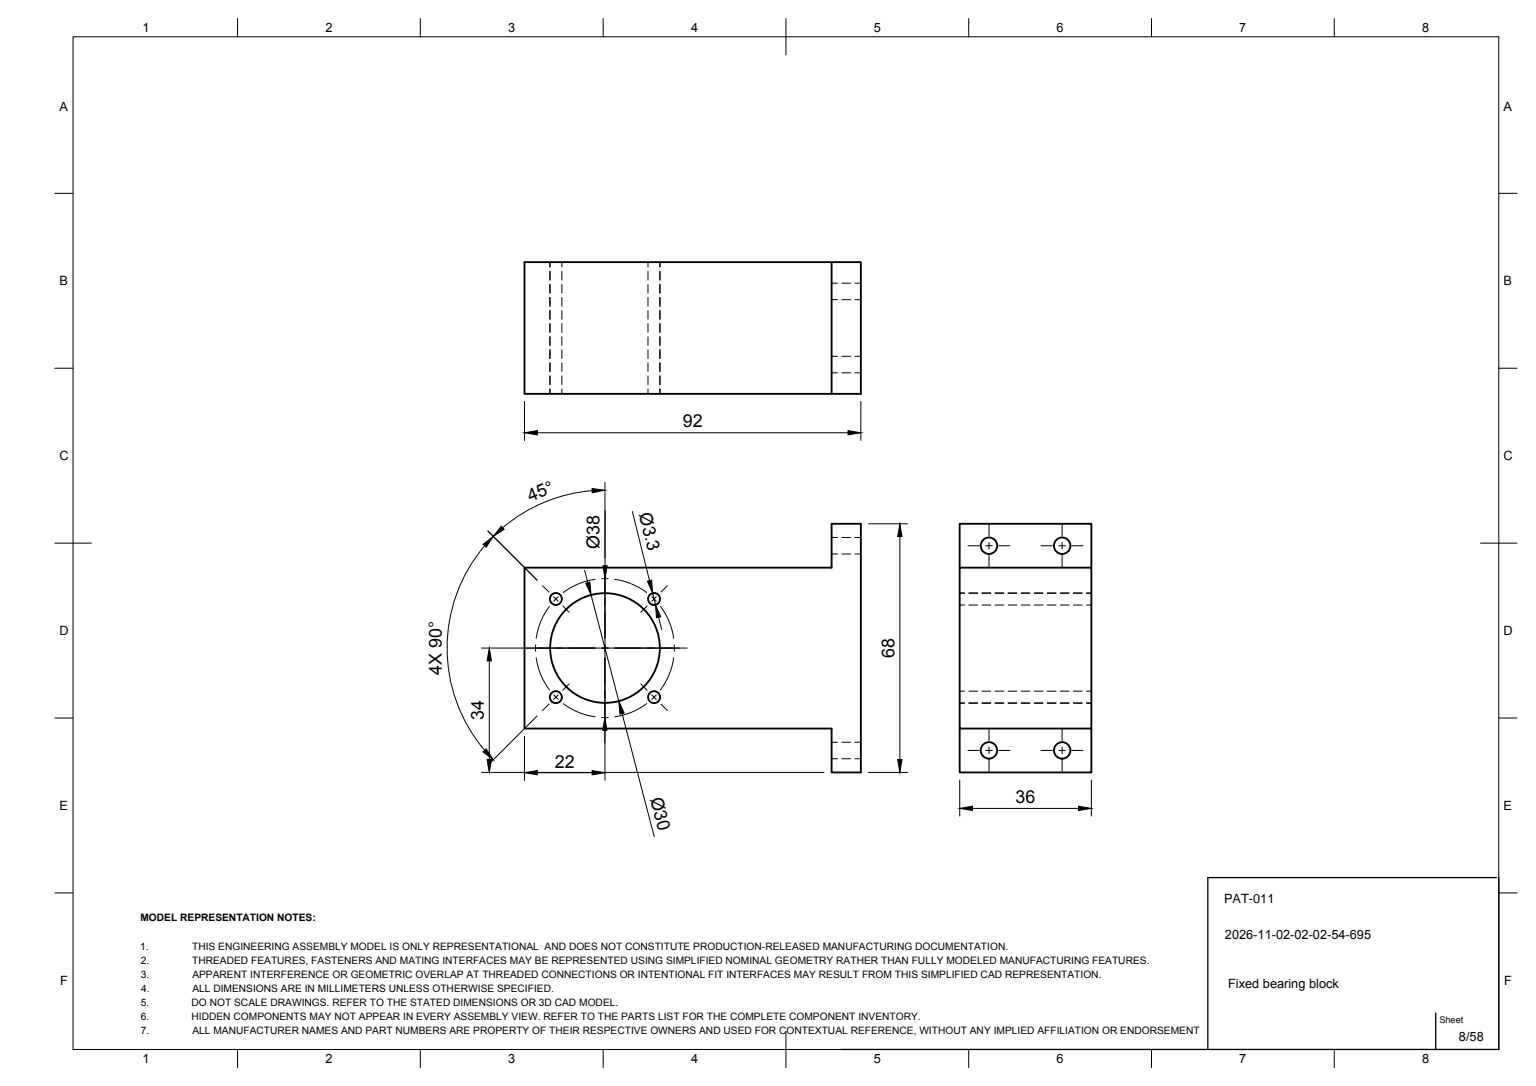
ISO-10303-21;
HEADER;
/* Generated by software containing ST-Developer
 * from STEP Tools, Inc. (www.steptools.com) 
 */

FILE_DESCRIPTION(
/* description */ ('Belt tension measurement rig'),
/* implementation_level */ '2;1');

FILE_NAME(
/* name */ 'Fixed bearing block.step',
/* time_stamp */ '2026-10-28T03:24:44-07:00',
/* author */ (''),
/* organization */ (''),
/* preprocessor_version */ 'ST-DEVELOPER v20.2',
/* originating_system */ 'Autodesk Translation Framework v15.17.0.0',
/* authorisation */ '');

FILE_SCHEMA (('AUTOMOTIVE_DESIGN { 1 0 10303 214 3 1 1 }'));
ENDSEC;

DATA;
#10=MECHANICAL_DESIGN_GEOMETRIC_PRESENTATION_REPRESENTATION('',(#695),#23587);
#585=SHAPE_REPRESENTATION_RELATIONSHIP('SRR','None',#23830,#640);
#640=ADVANCED_BREP_SHAPE_REPRESENTATION('',(#765),#23528);
#695=STYLED_ITEM('',(#24211),#765);
#765=MANIFOLD_SOLID_BREP('Body1',#12200);
#843=FACE_BOUND('',#2126,.T.);
#844=FACE_BOUND('',#2127,.T.);
#845=FACE_BOUND('',#2129,.T.);
#846=FACE_BOUND('',#2130,.T.);
#847=FACE_BOUND('',#2134,.T.);
#848=FACE_BOUND('',#2135,.T.);
#849=FACE_BOUND('',#2136,.T.);
#850=FACE_BOUND('',#2137,.T.);
#851=FACE_BOUND('',#2138,.T.);
#852=FACE_BOUND('',#2141,.T.);
#853=FACE_BOUND('',#2142,.T.);
#854=FACE_BOUND('',#2143,.T.);
#855=FACE_BOUND('',#2144,.T.);
#856=FACE_BOUND('',#2145,.T.);
#857=FACE_BOUND('',#2149,.T.);
#858=FACE_BOUND('',#2150,.T.);
#859=FACE_BOUND('',#2151,.T.);
#860=FACE_BOUND('',#2152,.T.);
#1069=PLANE('',#12983);
#1070=PLANE('',#12984);
#1071=PLANE('',#12985);
#1072=PLANE('',#12986);
#1073=PLANE('',#12987);
#1074=PLANE('',#12988);
#1075=PLANE('',#12989);
#1076=PLANE('',#12990);
#1077=PLANE('',#12991);
#1078=PLANE('',#12992);
#1398=FACE_OUTER_BOUND('',#2116,.T.);
#1399=FACE_OUTER_BOUND('',#2117,.T.);
#1400=FACE_OUTER_BOUND('',#2118,.T.);
#1401=FACE_OUTER_BOUND('',#2119,.T.);
#1402=FACE_OUTER_BOUND('',#2120,.T.);
#1403=FACE_OUTER_BOUND('',#2121,.T.);
#1404=FACE_OUTER_BOUND('',#2122,.T.);
#1405=FACE_OUTER_BOUND('',#2123,.T.);
#1406=FACE_OUTER_BOUND('',#2124,.T.);
#1407=FACE_OUTER_BOUND('',#2125,.T.);
#1408=FACE_OUTER_BOUND('',#2128,.T.);
#1409=FACE_OUTER_BOUND('',#2131,.T.);
#1410=FACE_OUTER_BOUND('',#2132,.T.);
#1411=FACE_OUTER_BOUND('',#2133,.T.);
#1412=FACE_OUTER_BOUND('',#2139,.T.);
#1413=FACE_OUTER_BOUND('',#2140,.T.);
#1414=FACE_OUTER_BOUND('',#2146,.T.);
#1415=FACE_OUTER_BOUND('',#2147,.T.);
#1416=FACE_OUTER_BOUND('',#2148,.T.);
#2116=EDGE_LOOP('',(#8094,#8095,#8096,#8097));
#2117=EDGE_LOOP('',(#8098,#8099,#8100,#8101));
#2118=EDGE_LOOP('',(#8102,#8103,#8104,#8105));
#2119=EDGE_LOOP('',(#8106,#8107,#8108,#8109));
#2120=EDGE_LOOP('',(#8110,#8111,#8112,#8113));
#2121=EDGE_LOOP('',(#8114,#8115,#8116,#8117));
#2122=EDGE_LOOP('',(#8118,#8119,#8120,#8121));
#2123=EDGE_LOOP('',(#8122,#8123,#8124,#8125));
#2124=EDGE_LOOP('',(#8126,#8127,#8128,#8129));
#2125=EDGE_LOOP('',(#8130,#8131,#8132,#8133));
#2126=EDGE_LOOP('',(#8134));
#2127=EDGE_LOOP('',(#8135));
#2128=EDGE_LOOP('',(#8136,#8137,#8138,#8139));
#2129=EDGE_LOOP('',(#8140));
#2130=EDGE_LOOP('',(#8141));
#2131=EDGE_LOOP('',(#8142,#8143,#8144,#8145));
#2132=EDGE_LOOP('',(#8146,#8147,#8148,#8149));
#2133=EDGE_LOOP('',(#8150,#8151,#8152,#8153,#8154,#8155,#8156,#8157));
#2134=EDGE_LOOP('',(#8158));
#2135=EDGE_LOOP('',(#8159));
#2136=EDGE_LOOP('',(#8160));
#2137=EDGE_LOOP('',(#8161));
#2138=EDGE_LOOP('',(#8162));
#2139=EDGE_LOOP('',(#8163,#8164,#8165,#8166));
#2140=EDGE_LOOP('',(#8167,#8168,#8169,#8170,#8171,#8172,#8173,#8174));
#2141=EDGE_LOOP('',(#8175));
#2142=EDGE_LOOP('',(#8176));
#2143=EDGE_LOOP('',(#8177));
#2144=EDGE_LOOP('',(#8178));
#2145=EDGE_LOOP('',(#8179));
#2146=EDGE_LOOP('',(#8180,#8181,#8182,#8183));
#2147=EDGE_LOOP('',(#8184,#8185,#8186,#8187));
#2148=EDGE_LOOP('',(#8188,#8189,#8190,#8191));
#2149=EDGE_LOOP('',(#8192));
#2150=EDGE_LOOP('',(#8193));
#2151=EDGE_LOOP('',(#8194));
#2152=EDGE_LOOP('',(#8195));
#3018=LINE('',#18736,#3769);
#3019=LINE('',#18742,#3770);
#3020=LINE('',#18748,#3771);
#3021=LINE('',#18754,#3772);
#3022=LINE('',#18760,#3773);
#3023=LINE('',#18766,#3774);
#3024=LINE('',#18772,#3775);
#3025=LINE('',#18778,#3776);
#3026=LINE('',#18784,#3777);
#3027=LINE('',#18789,#3778);
#3028=LINE('',#18791,#3779);
#3029=LINE('',#18793,#3780);
#3030=LINE('',#18794,#3781);
#3031=LINE('',#18798,#3782);
#3032=LINE('',#18800,#3783);
#3033=LINE('',#18802,#3784);
#3034=LINE('',#18803,#3785);
#3035=LINE('',#18806,#3786);
#3036=LINE('',#18808,#3787);
#3037=LINE('',#18809,#3788);
#3038=LINE('',#18812,#3789);
#3039=LINE('',#18814,#3790);
#3040=LINE('',#18815,#3791);
#3041=LINE('',#18818,#3792);
#3042=LINE('',#18820,#3793);
#3043=LINE('',#18821,#3794);
#3044=LINE('',#18822,#3795);
#3045=LINE('',#18825,#3796);
#3046=LINE('',#18826,#3797);
#3047=LINE('',#18829,#3798);
#3048=LINE('',#18830,#3799);
#3049=LINE('',#18831,#3800);
#3050=LINE('',#18833,#3801);
#3769=VECTOR('',#14731,0.165);
#3770=VECTOR('',#14738,0.165);
#3771=VECTOR('',#14745,0.165);
#3772=VECTOR('',#14752,0.165);
#3773=VECTOR('',#14759,1.5);
#3774=VECTOR('',#14766,0.225);
#3775=VECTOR('',#14773,0.225);
#3776=VECTOR('',#14780,0.225);
#3777=VECTOR('',#14787,0.225);
#3778=VECTOR('',#14792,1.);
#3779=VECTOR('',#14793,1.);
#3780=VECTOR('',#14794,1.);
#3781=VECTOR('',#14795,1.);
#3782=VECTOR('',#14798,1.);
#3783=VECTOR('',#14799,1.);
#3784=VECTOR('',#14800,1.);
#3785=VECTOR('',#14801,1.);
#3786=VECTOR('',#14804,1.);
#3787=VECTOR('',#14805,1.);
#3788=VECTOR('',#14806,1.);
#3789=VECTOR('',#14809,1.);
#3790=VECTOR('',#14810,1.);
#3791=VECTOR('',#14811,1.);
#3792=VECTOR('',#14814,1.);
#3793=VECTOR('',#14815,1.);
#3794=VECTOR('',#14816,1.);
#3795=VECTOR('',#14817,1.);
#3796=VECTOR('',#14820,1.);
#3797=VECTOR('',#14821,1.);
#3798=VECTOR('',#14824,1.);
#3799=VECTOR('',#14825,1.);
#3800=VECTOR('',#14826,1.);
#3801=VECTOR('',#14829,1.);
#4498=CIRCLE('',#12957,0.165);
#4499=CIRCLE('',#12958,0.165);
#4500=CIRCLE('',#12960,0.165);
#4501=CIRCLE('',#12961,0.165);
#4502=CIRCLE('',#12963,0.165);
#4503=CIRCLE('',#12964,0.165);
#4504=CIRCLE('',#12966,0.165);
#4505=CIRCLE('',#12967,0.165);
#4506=CIRCLE('',#12969,1.5);
#4507=CIRCLE('',#12970,1.5);
#4508=CIRCLE('',#12972,0.225);
#4509=CIRCLE('',#12973,0.225);
#4510=CIRCLE('',#12975,0.225);
#4511=CIRCLE('',#12976,0.225);
#4512=CIRCLE('',#12978,0.225);
#4513=CIRCLE('',#12979,0.225);
#4514=CIRCLE('',#12981,0.225);
#4515=CIRCLE('',#12982,0.225);
#5290=VERTEX_POINT('',#18733);
#5291=VERTEX_POINT('',#18735);
#5292=VERTEX_POINT('',#18739);
#5293=VERTEX_POINT('',#18741);
#5294=VERTEX_POINT('',#18745);
#5295=VERTEX_POINT('',#18747);
#5296=VERTEX_POINT('',#18751);
#5297=VERTEX_POINT('',#18753);
#5298=VERTEX_POINT('',#18757);
#5299=VERTEX_POINT('',#18759);
#5300=VERTEX_POINT('',#18763);
#5301=VERTEX_POINT('',#18765);
#5302=VERTEX_POINT('',#18769);
#5303=VERTEX_POINT('',#18771);
#5304=VERTEX_POINT('',#18775);
#5305=VERTEX_POINT('',#18777);
#5306=VERTEX_POINT('',#18781);
#5307=VERTEX_POINT('',#18783);
#5308=VERTEX_POINT('',#18787);
#5309=VERTEX_POINT('',#18788);
#5310=VERTEX_POINT('',#18790);
#5311=VERTEX_POINT('',#18792);
#5312=VERTEX_POINT('',#18796);
#5313=VERTEX_POINT('',#18797);
#5314=VERTEX_POINT('',#18799);
#5315=VERTEX_POINT('',#18801);
#5316=VERTEX_POINT('',#18805);
#5317=VERTEX_POINT('',#18807);
#5318=VERTEX_POINT('',#18811);
#5319=VERTEX_POINT('',#18813);
#5320=VERTEX_POINT('',#18817);
#5321=VERTEX_POINT('',#18819);
#5322=VERTEX_POINT('',#18824);
#5323=VERTEX_POINT('',#18828);
#6406=EDGE_CURVE('',#5290,#5290,#4498,.T.);
#6407=EDGE_CURVE('',#5290,#5291,#3018,.T.);
#6408=EDGE_CURVE('',#5291,#5291,#4499,.T.);
#6409=EDGE_CURVE('',#5292,#5292,#4500,.T.);
#6410=EDGE_CURVE('',#5292,#5293,#3019,.T.);
#6411=EDGE_CURVE('',#5293,#5293,#4501,.T.);
#6412=EDGE_CURVE('',#5294,#5294,#4502,.T.);
#6413=EDGE_CURVE('',#5294,#5295,#3020,.T.);
#6414=EDGE_CURVE('',#5295,#5295,#4503,.T.);
#6415=EDGE_CURVE('',#5296,#5296,#4504,.T.);
#6416=EDGE_CURVE('',#5296,#5297,#3021,.T.);
#6417=EDGE_CURVE('',#5297,#5297,#4505,.T.);
#6418=EDGE_CURVE('',#5298,#5298,#4506,.T.);
#6419=EDGE_CURVE('',#5298,#5299,#3022,.T.);
#6420=EDGE_CURVE('',#5299,#5299,#4507,.T.);
#6421=EDGE_CURVE('',#5300,#5300,#4508,.T.);
#6422=EDGE_CURVE('',#5300,#5301,#3023,.T.);
#6423=EDGE_CURVE('',#5301,#5301,#4509,.T.);
#6424=EDGE_CURVE('',#5302,#5302,#4510,.T.);
#6425=EDGE_CURVE('',#5302,#5303,#3024,.T.);
#6426=EDGE_CURVE('',#5303,#5303,#4511,.T.);
#6427=EDGE_CURVE('',#5304,#5304,#4512,.T.);
#6428=EDGE_CURVE('',#5304,#5305,#3025,.T.);
#6429=EDGE_CURVE('',#5305,#5305,#4513,.T.);
#6430=EDGE_CURVE('',#5306,#5306,#4514,.T.);
#6431=EDGE_CURVE('',#5306,#5307,#3026,.T.);
#6432=EDGE_CURVE('',#5307,#5307,#4515,.T.);
#6433=EDGE_CURVE('',#5308,#5309,#3027,.T.);
#6434=EDGE_CURVE('',#5310,#5308,#3028,.T.);
#6435=EDGE_CURVE('',#5310,#5311,#3029,.T.);
#6436=EDGE_CURVE('',#5309,#5311,#3030,.T.);
#6437=EDGE_CURVE('',#5312,#5313,#3031,.T.);
#6438=EDGE_CURVE('',#5314,#5312,#3032,.T.);
#6439=EDGE_CURVE('',#5315,#5314,#3033,.T.);
#6440=EDGE_CURVE('',#5313,#5315,#3034,.T.);
#6441=EDGE_CURVE('',#5315,#5316,#3035,.T.);
#6442=EDGE_CURVE('',#5317,#5314,#3036,.T.);
#6443=EDGE_CURVE('',#5316,#5317,#3037,.T.);
#6444=EDGE_CURVE('',#5318,#5310,#3038,.T.);
#6445=EDGE_CURVE('',#5318,#5319,#3039,.T.);
#6446=EDGE_CURVE('',#5311,#5319,#3040,.T.);
#6447=EDGE_CURVE('',#5308,#5320,#3041,.T.);
#6448=EDGE_CURVE('',#5321,#5320,#3042,.T.);
#6449=EDGE_CURVE('',#5313,#5321,#3043,.T.);
#6450=EDGE_CURVE('',#5316,#5318,#3044,.T.);
#6451=EDGE_CURVE('',#5309,#5322,#3045,.T.);
#6452=EDGE_CURVE('',#5320,#5322,#3046,.T.);
#6453=EDGE_CURVE('',#5312,#5323,#3047,.T.);
#6454=EDGE_CURVE('',#5322,#5323,#3048,.T.);
#6455=EDGE_CURVE('',#5319,#5317,#3049,.T.);
#6456=EDGE_CURVE('',#5323,#5321,#3050,.T.);
#8094=ORIENTED_EDGE('',*,*,#6406,.F.);
#8095=ORIENTED_EDGE('',*,*,#6407,.T.);
#8096=ORIENTED_EDGE('',*,*,#6408,.F.);
#8097=ORIENTED_EDGE('',*,*,#6407,.F.);
#8098=ORIENTED_EDGE('',*,*,#6409,.F.);
#8099=ORIENTED_EDGE('',*,*,#6410,.T.);
#8100=ORIENTED_EDGE('',*,*,#6411,.F.);
#8101=ORIENTED_EDGE('',*,*,#6410,.F.);
#8102=ORIENTED_EDGE('',*,*,#6412,.F.);
#8103=ORIENTED_EDGE('',*,*,#6413,.T.);
#8104=ORIENTED_EDGE('',*,*,#6414,.F.);
#8105=ORIENTED_EDGE('',*,*,#6413,.F.);
#8106=ORIENTED_EDGE('',*,*,#6415,.F.);
#8107=ORIENTED_EDGE('',*,*,#6416,.T.);
#8108=ORIENTED_EDGE('',*,*,#6417,.F.);
#8109=ORIENTED_EDGE('',*,*,#6416,.F.);
#8110=ORIENTED_EDGE('',*,*,#6418,.F.);
#8111=ORIENTED_EDGE('',*,*,#6419,.T.);
#8112=ORIENTED_EDGE('',*,*,#6420,.F.);
#8113=ORIENTED_EDGE('',*,*,#6419,.F.);
#8114=ORIENTED_EDGE('',*,*,#6421,.F.);
#8115=ORIENTED_EDGE('',*,*,#6422,.T.);
#8116=ORIENTED_EDGE('',*,*,#6423,.F.);
#8117=ORIENTED_EDGE('',*,*,#6422,.F.);
#8118=ORIENTED_EDGE('',*,*,#6424,.F.);
#8119=ORIENTED_EDGE('',*,*,#6425,.T.);
#8120=ORIENTED_EDGE('',*,*,#6426,.F.);
#8121=ORIENTED_EDGE('',*,*,#6425,.F.);
#8122=ORIENTED_EDGE('',*,*,#6427,.F.);
#8123=ORIENTED_EDGE('',*,*,#6428,.T.);
#8124=ORIENTED_EDGE('',*,*,#6429,.F.);
#8125=ORIENTED_EDGE('',*,*,#6428,.F.);
#8126=ORIENTED_EDGE('',*,*,#6430,.F.);
#8127=ORIENTED_EDGE('',*,*,#6431,.T.);
#8128=ORIENTED_EDGE('',*,*,#6432,.F.);
#8129=ORIENTED_EDGE('',*,*,#6431,.F.);
#8130=ORIENTED_EDGE('',*,*,#6433,.F.);
#8131=ORIENTED_EDGE('',*,*,#6434,.F.);
#8132=ORIENTED_EDGE('',*,*,#6435,.T.);
#8133=ORIENTED_EDGE('',*,*,#6436,.F.);
#8134=ORIENTED_EDGE('',*,*,#6423,.T.);
#8135=ORIENTED_EDGE('',*,*,#6432,.T.);
#8136=ORIENTED_EDGE('',*,*,#6437,.F.);
#8137=ORIENTED_EDGE('',*,*,#6438,.F.);
#8138=ORIENTED_EDGE('',*,*,#6439,.F.);
#8139=ORIENTED_EDGE('',*,*,#6440,.F.);
#8140=ORIENTED_EDGE('',*,*,#6426,.T.);
#8141=ORIENTED_EDGE('',*,*,#6429,.T.);
#8142=ORIENTED_EDGE('',*,*,#6441,.F.);
#8143=ORIENTED_EDGE('',*,*,#6439,.T.);
#8144=ORIENTED_EDGE('',*,*,#6442,.F.);
#8145=ORIENTED_EDGE('',*,*,#6443,.F.);
#8146=ORIENTED_EDGE('',*,*,#6444,.F.);
#8147=ORIENTED_EDGE('',*,*,#6445,.T.);
#8148=ORIENTED_EDGE('',*,*,#6446,.F.);
#8149=ORIENTED_EDGE('',*,*,#6435,.F.);
#8150=ORIENTED_EDGE('',*,*,#6447,.T.);
#8151=ORIENTED_EDGE('',*,*,#6448,.F.);
#8152=ORIENTED_EDGE('',*,*,#6449,.F.);
#8153=ORIENTED_EDGE('',*,*,#6440,.T.);
#8154=ORIENTED_EDGE('',*,*,#6441,.T.);
#8155=ORIENTED_EDGE('',*,*,#6450,.T.);
#8156=ORIENTED_EDGE('',*,*,#6444,.T.);
#8157=ORIENTED_EDGE('',*,*,#6434,.T.);
#8158=ORIENTED_EDGE('',*,*,#6418,.T.);
#8159=ORIENTED_EDGE('',*,*,#6415,.T.);
#8160=ORIENTED_EDGE('',*,*,#6412,.T.);
#8161=ORIENTED_EDGE('',*,*,#6409,.T.);
#8162=ORIENTED_EDGE('',*,*,#6406,.T.);
#8163=ORIENTED_EDGE('',*,*,#6433,.T.);
#8164=ORIENTED_EDGE('',*,*,#6451,.T.);
#8165=ORIENTED_EDGE('',*,*,#6452,.F.);
#8166=ORIENTED_EDGE('',*,*,#6447,.F.);
#8167=ORIENTED_EDGE('',*,*,#6453,.T.);
#8168=ORIENTED_EDGE('',*,*,#6454,.F.);
#8169=ORIENTED_EDGE('',*,*,#6451,.F.);
#8170=ORIENTED_EDGE('',*,*,#6436,.T.);
#8171=ORIENTED_EDGE('',*,*,#6446,.T.);
#8172=ORIENTED_EDGE('',*,*,#6455,.T.);
#8173=ORIENTED_EDGE('',*,*,#6442,.T.);
#8174=ORIENTED_EDGE('',*,*,#6438,.T.);
#8175=ORIENTED_EDGE('',*,*,#6420,.T.);
#8176=ORIENTED_EDGE('',*,*,#6417,.T.);
#8177=ORIENTED_EDGE('',*,*,#6414,.T.);
#8178=ORIENTED_EDGE('',*,*,#6411,.T.);
#8179=ORIENTED_EDGE('',*,*,#6408,.T.);
#8180=ORIENTED_EDGE('',*,*,#6437,.T.);
#8181=ORIENTED_EDGE('',*,*,#6449,.T.);
#8182=ORIENTED_EDGE('',*,*,#6456,.F.);
#8183=ORIENTED_EDGE('',*,*,#6453,.F.);
#8184=ORIENTED_EDGE('',*,*,#6456,.T.);
#8185=ORIENTED_EDGE('',*,*,#6448,.T.);
#8186=ORIENTED_EDGE('',*,*,#6452,.T.);
#8187=ORIENTED_EDGE('',*,*,#6454,.T.);
#8188=ORIENTED_EDGE('',*,*,#6455,.F.);
#8189=ORIENTED_EDGE('',*,*,#6445,.F.);
#8190=ORIENTED_EDGE('',*,*,#6450,.F.);
#8191=ORIENTED_EDGE('',*,*,#6443,.T.);
#8192=ORIENTED_EDGE('',*,*,#6421,.T.);
#8193=ORIENTED_EDGE('',*,*,#6424,.T.);
#8194=ORIENTED_EDGE('',*,*,#6427,.T.);
#8195=ORIENTED_EDGE('',*,*,#6430,.T.);
#11172=CYLINDRICAL_SURFACE('',#12956,0.165);
#11173=CYLINDRICAL_SURFACE('',#12959,0.165);
#11174=CYLINDRICAL_SURFACE('',#12962,0.165);
#11175=CYLINDRICAL_SURFACE('',#12965,0.165);
#11176=CYLINDRICAL_SURFACE('',#12968,1.5);
#11177=CYLINDRICAL_SURFACE('',#12971,0.225);
#11178=CYLINDRICAL_SURFACE('',#12974,0.225);
#11179=CYLINDRICAL_SURFACE('',#12977,0.225);
#11180=CYLINDRICAL_SURFACE('',#12980,0.225);
#11539=ADVANCED_FACE('',(#1398),#11172,.F.);
#11540=ADVANCED_FACE('',(#1399),#11173,.F.);
#11541=ADVANCED_FACE('',(#1400),#11174,.F.);
#11542=ADVANCED_FACE('',(#1401),#11175,.F.);
#11543=ADVANCED_FACE('',(#1402),#11176,.F.);
#11544=ADVANCED_FACE('',(#1403),#11177,.F.);
#11545=ADVANCED_FACE('',(#1404),#11178,.F.);
#11546=ADVANCED_FACE('',(#1405),#11179,.F.);
#11547=ADVANCED_FACE('',(#1406),#11180,.F.);
#11548=ADVANCED_FACE('',(#1407,#843,#844),#1069,.T.);
#11549=ADVANCED_FACE('',(#1408,#845,#846),#1070,.T.);
#11550=ADVANCED_FACE('',(#1409),#1071,.T.);
#11551=ADVANCED_FACE('',(#1410),#1072,.T.);
#11552=ADVANCED_FACE('',(#1411,#847,#848,#849,#850,#851),#1073,.T.);
#11553=ADVANCED_FACE('',(#1412),#1074,.T.);
#11554=ADVANCED_FACE('',(#1413,#852,#853,#854,#855,#856),#1075,.T.);
#11555=ADVANCED_FACE('',(#1414),#1076,.T.);
#11556=ADVANCED_FACE('',(#1415),#1077,.T.);
#11557=ADVANCED_FACE('',(#1416,#857,#858,#859,#860),#1078,.F.);
#12200=CLOSED_SHELL('',(#11539,#11540,#11541,#11542,#11543,#11544,#11545,
#11546,#11547,#11548,#11549,#11550,#11551,#11552,#11553,#11554,#11555,#11556,
#11557));
#12955=AXIS2_PLACEMENT_3D('',#18731,#14725,#14726);
#12956=AXIS2_PLACEMENT_3D('',#18732,#14727,#14728);
#12957=AXIS2_PLACEMENT_3D('',#18734,#14729,#14730);
#12958=AXIS2_PLACEMENT_3D('',#18737,#14732,#14733);
#12959=AXIS2_PLACEMENT_3D('',#18738,#14734,#14735);
#12960=AXIS2_PLACEMENT_3D('',#18740,#14736,#14737);
#12961=AXIS2_PLACEMENT_3D('',#18743,#14739,#14740);
#12962=AXIS2_PLACEMENT_3D('',#18744,#14741,#14742);
#12963=AXIS2_PLACEMENT_3D('',#18746,#14743,#14744);
#12964=AXIS2_PLACEMENT_3D('',#18749,#14746,#14747);
#12965=AXIS2_PLACEMENT_3D('',#18750,#14748,#14749);
#12966=AXIS2_PLACEMENT_3D('',#18752,#14750,#14751);
#12967=AXIS2_PLACEMENT_3D('',#18755,#14753,#14754);
#12968=AXIS2_PLACEMENT_3D('',#18756,#14755,#14756);
#12969=AXIS2_PLACEMENT_3D('',#18758,#14757,#14758);
#12970=AXIS2_PLACEMENT_3D('',#18761,#14760,#14761);
#12971=AXIS2_PLACEMENT_3D('',#18762,#14762,#14763);
#12972=AXIS2_PLACEMENT_3D('',#18764,#14764,#14765);
#12973=AXIS2_PLACEMENT_3D('',#18767,#14767,#14768);
#12974=AXIS2_PLACEMENT_3D('',#18768,#14769,#14770);
#12975=AXIS2_PLACEMENT_3D('',#18770,#14771,#14772);
#12976=AXIS2_PLACEMENT_3D('',#18773,#14774,#14775);
#12977=AXIS2_PLACEMENT_3D('',#18774,#14776,#14777);
#12978=AXIS2_PLACEMENT_3D('',#18776,#14778,#14779);
#12979=AXIS2_PLACEMENT_3D('',#18779,#14781,#14782);
#12980=AXIS2_PLACEMENT_3D('',#18780,#14783,#14784);
#12981=AXIS2_PLACEMENT_3D('',#18782,#14785,#14786);
#12982=AXIS2_PLACEMENT_3D('',#18785,#14788,#14789);
#12983=AXIS2_PLACEMENT_3D('',#18786,#14790,#14791);
#12984=AXIS2_PLACEMENT_3D('',#18795,#14796,#14797);
#12985=AXIS2_PLACEMENT_3D('',#18804,#14802,#14803);
#12986=AXIS2_PLACEMENT_3D('',#18810,#14807,#14808);
#12987=AXIS2_PLACEMENT_3D('',#18816,#14812,#14813);
#12988=AXIS2_PLACEMENT_3D('',#18823,#14818,#14819);
#12989=AXIS2_PLACEMENT_3D('',#18827,#14822,#14823);
#12990=AXIS2_PLACEMENT_3D('',#18832,#14827,#14828);
#12991=AXIS2_PLACEMENT_3D('',#18834,#14830,#14831);
#12992=AXIS2_PLACEMENT_3D('',#18835,#14832,#14833);
#14725=DIRECTION('axis',(0.,0.,1.));
#14726=DIRECTION('refdir',(1.,0.,0.));
#14727=DIRECTION('center_axis',(0.,1.,0.));
#14728=DIRECTION('ref_axis',(1.,0.,0.));
#14729=DIRECTION('center_axis',(0.,1.,0.));
#14730=DIRECTION('ref_axis',(1.,0.,0.));
#14731=DIRECTION('',(0.,1.,0.));
#14732=DIRECTION('center_axis',(0.,-1.,0.));
#14733=DIRECTION('ref_axis',(1.,0.,0.));
#14734=DIRECTION('center_axis',(0.,1.,0.));
#14735=DIRECTION('ref_axis',(1.,0.,0.));
#14736=DIRECTION('center_axis',(0.,1.,0.));
#14737=DIRECTION('ref_axis',(1.,0.,0.));
#14738=DIRECTION('',(0.,1.,0.));
#14739=DIRECTION('center_axis',(0.,-1.,0.));
#14740=DIRECTION('ref_axis',(1.,0.,0.));
#14741=DIRECTION('center_axis',(0.,1.,0.));
#14742=DIRECTION('ref_axis',(1.,0.,0.));
#14743=DIRECTION('center_axis',(0.,1.,0.));
#14744=DIRECTION('ref_axis',(1.,0.,0.));
#14745=DIRECTION('',(0.,1.,0.));
#14746=DIRECTION('center_axis',(0.,-1.,0.));
#14747=DIRECTION('ref_axis',(1.,0.,0.));
#14748=DIRECTION('center_axis',(0.,1.,0.));
#14749=DIRECTION('ref_axis',(1.,0.,0.));
#14750=DIRECTION('center_axis',(0.,1.,0.));
#14751=DIRECTION('ref_axis',(1.,0.,0.));
#14752=DIRECTION('',(0.,1.,0.));
#14753=DIRECTION('center_axis',(0.,-1.,0.));
#14754=DIRECTION('ref_axis',(1.,0.,0.));
#14755=DIRECTION('center_axis',(0.,1.,0.));
#14756=DIRECTION('ref_axis',(1.,0.,0.));
#14757=DIRECTION('center_axis',(0.,1.,0.));
#14758=DIRECTION('ref_axis',(1.,0.,0.));
#14759=DIRECTION('',(0.,1.,0.));
#14760=DIRECTION('center_axis',(0.,-1.,0.));
#14761=DIRECTION('ref_axis',(1.,0.,0.));
#14762=DIRECTION('center_axis',(0.,0.,1.));
#14763=DIRECTION('ref_axis',(1.,0.,0.));
#14764=DIRECTION('center_axis',(0.,0.,1.));
#14765=DIRECTION('ref_axis',(1.,0.,0.));
#14766=DIRECTION('',(0.,0.,1.));
#14767=DIRECTION('center_axis',(0.,0.,-1.));
#14768=DIRECTION('ref_axis',(1.,0.,0.));
#14769=DIRECTION('center_axis',(0.,0.,1.));
#14770=DIRECTION('ref_axis',(1.,0.,0.));
#14771=DIRECTION('center_axis',(0.,0.,1.));
#14772=DIRECTION('ref_axis',(1.,0.,0.));
#14773=DIRECTION('',(0.,0.,1.));
#14774=DIRECTION('center_axis',(0.,0.,-1.));
#14775=DIRECTION('ref_axis',(1.,0.,0.));
#14776=DIRECTION('center_axis',(0.,0.,1.));
#14777=DIRECTION('ref_axis',(1.,0.,0.));
#14778=DIRECTION('center_axis',(0.,0.,1.));
#14779=DIRECTION('ref_axis',(1.,0.,0.));
#14780=DIRECTION('',(0.,0.,1.));
#14781=DIRECTION('center_axis',(0.,0.,-1.));
#14782=DIRECTION('ref_axis',(1.,0.,0.));
#14783=DIRECTION('center_axis',(0.,0.,1.));
#14784=DIRECTION('ref_axis',(1.,0.,0.));
#14785=DIRECTION('center_axis',(0.,0.,1.));
#14786=DIRECTION('ref_axis',(1.,0.,0.));
#14787=DIRECTION('',(0.,0.,1.));
#14788=DIRECTION('center_axis',(0.,0.,-1.));
#14789=DIRECTION('ref_axis',(1.,0.,0.));
#14790=DIRECTION('center_axis',(0.,0.,1.));
#14791=DIRECTION('ref_axis',(1.,0.,0.));
#14792=DIRECTION('',(0.,1.,0.));
#14793=DIRECTION('',(-1.,0.,0.));
#14794=DIRECTION('',(0.,1.,0.));
#14795=DIRECTION('',(1.,0.,0.));
#14796=DIRECTION('center_axis',(0.,0.,1.));
#14797=DIRECTION('ref_axis',(1.,0.,0.));
#14798=DIRECTION('',(0.,-1.,0.));
#14799=DIRECTION('',(1.,0.,0.));
#14800=DIRECTION('',(0.,1.,0.));
#14801=DIRECTION('',(-1.,0.,0.));
#14802=DIRECTION('center_axis',(-1.,0.,0.));
#14803=DIRECTION('ref_axis',(0.,0.,1.));
#14804=DIRECTION('',(0.,0.,-1.));
#14805=DIRECTION('',(0.,0.,1.));
#14806=DIRECTION('',(0.,1.,0.));
#14807=DIRECTION('center_axis',(1.,0.,0.));
#14808=DIRECTION('ref_axis',(0.,0.,-1.));
#14809=DIRECTION('',(0.,0.,1.));
#14810=DIRECTION('',(0.,1.,0.));
#14811=DIRECTION('',(0.,0.,-1.));
#14812=DIRECTION('center_axis',(0.,-1.,0.));
#14813=DIRECTION('ref_axis',(1.,0.,0.));
#14814=DIRECTION('',(0.,0.,1.));
#14815=DIRECTION('',(1.,0.,0.));
#14816=DIRECTION('',(0.,0.,1.));
#14817=DIRECTION('',(1.,0.,0.));
#14818=DIRECTION('center_axis',(1.,0.,0.));
#14819=DIRECTION('ref_axis',(0.,1.,0.));
#14820=DIRECTION('',(0.,0.,1.));
#14821=DIRECTION('',(0.,1.,0.));
#14822=DIRECTION('center_axis',(0.,1.,0.));
#14823=DIRECTION('ref_axis',(-1.,0.,0.));
#14824=DIRECTION('',(0.,0.,1.));
#14825=DIRECTION('',(-1.,0.,0.));
#14826=DIRECTION('',(-1.,0.,0.));
#14827=DIRECTION('center_axis',(-1.,0.,0.));
#14828=DIRECTION('ref_axis',(0.,-1.,0.));
#14829=DIRECTION('',(0.,-1.,0.));
#14830=DIRECTION('center_axis',(0.,0.,1.));
#14831=DIRECTION('ref_axis',(1.,0.,0.));
#14832=DIRECTION('center_axis',(0.,0.,1.));
#14833=DIRECTION('ref_axis',(1.,0.,0.));
#18731=CARTESIAN_POINT('',(0.,0.,0.));
#18732=CARTESIAN_POINT('Origin',(-1.34350288425444,-1.9,5.65649711574556));
#18733=CARTESIAN_POINT('',(-1.50850288425444,-1.8,5.65649711574556));
#18734=CARTESIAN_POINT('Origin',(-1.34350288425444,-1.8,5.65649711574556));
#18735=CARTESIAN_POINT('',(-1.50850288425444,1.8,5.65649711574556));
#18736=CARTESIAN_POINT('',(-1.50850288425444,-1.9,5.65649711574556));
#18737=CARTESIAN_POINT('Origin',(-1.34350288425444,1.8,5.65649711574556));
#18738=CARTESIAN_POINT('Origin',(-1.34350288425444,-1.9,8.34350288425444));
#18739=CARTESIAN_POINT('',(-1.50850288425444,-1.8,8.34350288425444));
#18740=CARTESIAN_POINT('Origin',(-1.34350288425444,-1.8,8.34350288425444));
#18741=CARTESIAN_POINT('',(-1.50850288425444,1.8,8.34350288425444));
#18742=CARTESIAN_POINT('',(-1.50850288425444,-1.9,8.34350288425444));
#18743=CARTESIAN_POINT('Origin',(-1.34350288425444,1.8,8.34350288425444));
#18744=CARTESIAN_POINT('Origin',(1.34350288425444,-1.9,8.34350288425444));
#18745=CARTESIAN_POINT('',(1.17850288425444,-1.8,8.34350288425444));
#18746=CARTESIAN_POINT('Origin',(1.34350288425444,-1.8,8.34350288425444));
#18747=CARTESIAN_POINT('',(1.17850288425444,1.8,8.34350288425444));
#18748=CARTESIAN_POINT('',(1.17850288425444,-1.9,8.34350288425444));
#18749=CARTESIAN_POINT('Origin',(1.34350288425444,1.8,8.34350288425444));
#18750=CARTESIAN_POINT('Origin',(1.34350288425444,-1.9,5.65649711574556));
#18751=CARTESIAN_POINT('',(1.17850288425444,-1.8,5.65649711574556));
#18752=CARTESIAN_POINT('Origin',(1.34350288425444,-1.8,5.65649711574556));
#18753=CARTESIAN_POINT('',(1.17850288425444,1.8,5.65649711574556));
#18754=CARTESIAN_POINT('',(1.17850288425444,-1.9,5.65649711574556));
#18755=CARTESIAN_POINT('Origin',(1.34350288425444,1.8,5.65649711574556));
#18756=CARTESIAN_POINT('Origin',(0.,-1.9,7.));
#18757=CARTESIAN_POINT('',(-1.5,-1.8,7.));
#18758=CARTESIAN_POINT('Origin',(0.,-1.8,7.));
#18759=CARTESIAN_POINT('',(-1.5,1.8,7.));
#18760=CARTESIAN_POINT('',(-1.5,-1.9,7.));
#18761=CARTESIAN_POINT('Origin',(0.,1.8,7.));
#18762=CARTESIAN_POINT('Origin',(2.8,-1.,-0.1));
#18763=CARTESIAN_POINT('',(2.575,-1.,0.));
#18764=CARTESIAN_POINT('Origin',(2.8,-1.,0.));
#18765=CARTESIAN_POINT('',(2.575,-1.,0.8));
#18766=CARTESIAN_POINT('',(2.575,-1.,-0.1));
#18767=CARTESIAN_POINT('Origin',(2.8,-1.,0.8));
#18768=CARTESIAN_POINT('Origin',(-2.8,1.,-0.1));
#18769=CARTESIAN_POINT('',(-3.025,1.,0.));
#18770=CARTESIAN_POINT('Origin',(-2.8,1.,0.));
#18771=CARTESIAN_POINT('',(-3.025,1.,0.8));
#18772=CARTESIAN_POINT('',(-3.025,1.,-0.1));
#18773=CARTESIAN_POINT('Origin',(-2.8,1.,0.8));
#18774=CARTESIAN_POINT('Origin',(-2.8,-1.,-0.1));
#18775=CARTESIAN_POINT('',(-3.025,-1.,0.));
#18776=CARTESIAN_POINT('Origin',(-2.8,-1.,0.));
#18777=CARTESIAN_POINT('',(-3.025,-1.,0.8));
#18778=CARTESIAN_POINT('',(-3.025,-1.,-0.1));
#18779=CARTESIAN_POINT('Origin',(-2.8,-1.,0.8));
#18780=CARTESIAN_POINT('Origin',(2.8,1.,-0.1));
#18781=CARTESIAN_POINT('',(2.575,1.,0.));
#18782=CARTESIAN_POINT('Origin',(2.8,1.,0.));
#18783=CARTESIAN_POINT('',(2.575,1.,0.8));
#18784=CARTESIAN_POINT('',(2.575,1.,-0.1));
#18785=CARTESIAN_POINT('Origin',(2.8,1.,0.8));
#18786=CARTESIAN_POINT('Origin',(-3.4,-1.8,0.8));
#18787=CARTESIAN_POINT('',(2.2,-1.8,0.8));
#18788=CARTESIAN_POINT('',(2.2,1.8,0.8));
#18789=CARTESIAN_POINT('',(2.2,-1.8,0.8));
#18790=CARTESIAN_POINT('',(3.4,-1.8,0.8));
#18791=CARTESIAN_POINT('',(3.4,-1.8,0.8));
#18792=CARTESIAN_POINT('',(3.4,1.8,0.8));
#18793=CARTESIAN_POINT('',(3.4,-1.8,0.8));
#18794=CARTESIAN_POINT('',(3.4,1.8,0.8));
#18795=CARTESIAN_POINT('Origin',(-3.4,-1.8,0.8));
#18796=CARTESIAN_POINT('',(-2.2,1.8,0.8));
#18797=CARTESIAN_POINT('',(-2.2,-1.8,0.8));
#18798=CARTESIAN_POINT('',(-2.2,0.,0.8));
#18799=CARTESIAN_POINT('',(-3.4,1.8,0.8));
#18800=CARTESIAN_POINT('',(3.4,1.8,0.8));
#18801=CARTESIAN_POINT('',(-3.4,-1.8,0.8));
#18802=CARTESIAN_POINT('',(-3.4,-1.8,0.8));
#18803=CARTESIAN_POINT('',(3.4,-1.8,0.8));
#18804=CARTESIAN_POINT('Origin',(-3.4,-1.8,0.));
#18805=CARTESIAN_POINT('',(-3.4,-1.8,0.));
#18806=CARTESIAN_POINT('',(-3.4,-1.8,0.8));
#18807=CARTESIAN_POINT('',(-3.4,1.8,0.));
#18808=CARTESIAN_POINT('',(-3.4,1.8,0.8));
#18809=CARTESIAN_POINT('',(-3.4,-1.8,0.));
#18810=CARTESIAN_POINT('Origin',(3.4,-1.8,0.8));
#18811=CARTESIAN_POINT('',(3.4,-1.8,0.));
#18812=CARTESIAN_POINT('',(3.4,-1.8,0.));
#18813=CARTESIAN_POINT('',(3.4,1.8,0.));
#18814=CARTESIAN_POINT('',(3.4,-1.8,0.));
#18815=CARTESIAN_POINT('',(3.4,1.8,0.));
#18816=CARTESIAN_POINT('Origin',(-2.2,-1.8,0.));
#18817=CARTESIAN_POINT('',(2.2,-1.8,9.2));
#18818=CARTESIAN_POINT('',(2.2,-1.8,0.));
#18819=CARTESIAN_POINT('',(-2.2,-1.8,9.2));
#18820=CARTESIAN_POINT('',(-2.2,-1.8,9.2));
#18821=CARTESIAN_POINT('',(-2.2,-1.8,0.));
#18822=CARTESIAN_POINT('',(-3.4,-1.8,0.));
#18823=CARTESIAN_POINT('Origin',(2.2,-1.8,0.));
#18824=CARTESIAN_POINT('',(2.2,1.8,9.2));
#18825=CARTESIAN_POINT('',(2.2,1.8,0.));
#18826=CARTESIAN_POINT('',(2.2,-1.8,9.2));
#18827=CARTESIAN_POINT('Origin',(2.2,1.8,0.));
#18828=CARTESIAN_POINT('',(-2.2,1.8,9.2));
#18829=CARTESIAN_POINT('',(-2.2,1.8,0.));
#18830=CARTESIAN_POINT('',(2.2,1.8,9.2));
#18831=CARTESIAN_POINT('',(-3.4,1.8,0.));
#18832=CARTESIAN_POINT('Origin',(-2.2,1.8,0.));
#18833=CARTESIAN_POINT('',(-2.2,1.8,9.2));
#18834=CARTESIAN_POINT('Origin',(0.,0.,9.2));
#18835=CARTESIAN_POINT('Origin',(0.,0.,0.));
#23463=UNCERTAINTY_MEASURE_WITH_UNIT(LENGTH_MEASURE(0.001),#23588,
'DISTANCE_ACCURACY_VALUE',
'Maximum model space distance between geometric entities at asserted c
onnectivities');
#23522=UNCERTAINTY_MEASURE_WITH_UNIT(LENGTH_MEASURE(0.001),#23588,
'DISTANCE_ACCURACY_VALUE',
'Maximum model space distance between geometric entities at asserted c
onnectivities');
#23528=(
GEOMETRIC_REPRESENTATION_CONTEXT(3)
GLOBAL_UNCERTAINTY_ASSIGNED_CONTEXT((#23463))
GLOBAL_UNIT_ASSIGNED_CONTEXT((#23588,#23590,#23591))
REPRESENTATION_CONTEXT('','3D')
);
#23587=(
GEOMETRIC_REPRESENTATION_CONTEXT(3)
GLOBAL_UNCERTAINTY_ASSIGNED_CONTEXT((#23522))
GLOBAL_UNIT_ASSIGNED_CONTEXT((#23588,#23590,#23591))
REPRESENTATION_CONTEXT('','3D')
);
#23588=(
LENGTH_UNIT()
NAMED_UNIT(*)
SI_UNIT(.CENTI.,.METRE.)
);
#23590=(
NAMED_UNIT(*)
PLANE_ANGLE_UNIT()
SI_UNIT($,.RADIAN.)
);
#23591=(
NAMED_UNIT(*)
SI_UNIT($,.STERADIAN.)
SOLID_ANGLE_UNIT()
);
#23597=SHAPE_DEFINITION_REPRESENTATION(#23661,#23830);
#23661=PRODUCT_DEFINITION_SHAPE('',$,#23895);
#23830=SHAPE_REPRESENTATION('',(#12955),#23528);
#23889=PRODUCT_DEFINITION_CONTEXT('part definition',#24083,'design');
#23895=PRODUCT_DEFINITION('Fixed bearing block','Fixed bearing block',#23959,
#23889);
#23959=PRODUCT_DEFINITION_FORMATION('',$,#24090);
#24083=APPLICATION_CONTEXT(
'Core Data for Automotive Mechanical Design Process');
#24084=PRODUCT_CONTEXT('part definition',#24083,'mechanical');
#24090=PRODUCT('Fixed bearing block','Fixed bearing block',
'Fixed bearing block',(#24084));
#24205=COLOUR_RGB('Grey',0.48,0.52,0.57);
#24206=FILL_AREA_STYLE_COLOUR('',#24205);
#24207=FILL_AREA_STYLE('',(#24206));
#24208=SURFACE_STYLE_FILL_AREA(#24207);
#24209=SURFACE_SIDE_STYLE('',(#24208));
#24210=SURFACE_STYLE_USAGE(.BOTH.,#24209);
#24211=PRESENTATION_STYLE_ASSIGNMENT((#24210));
ENDSEC;
END-ISO-10303-21;
